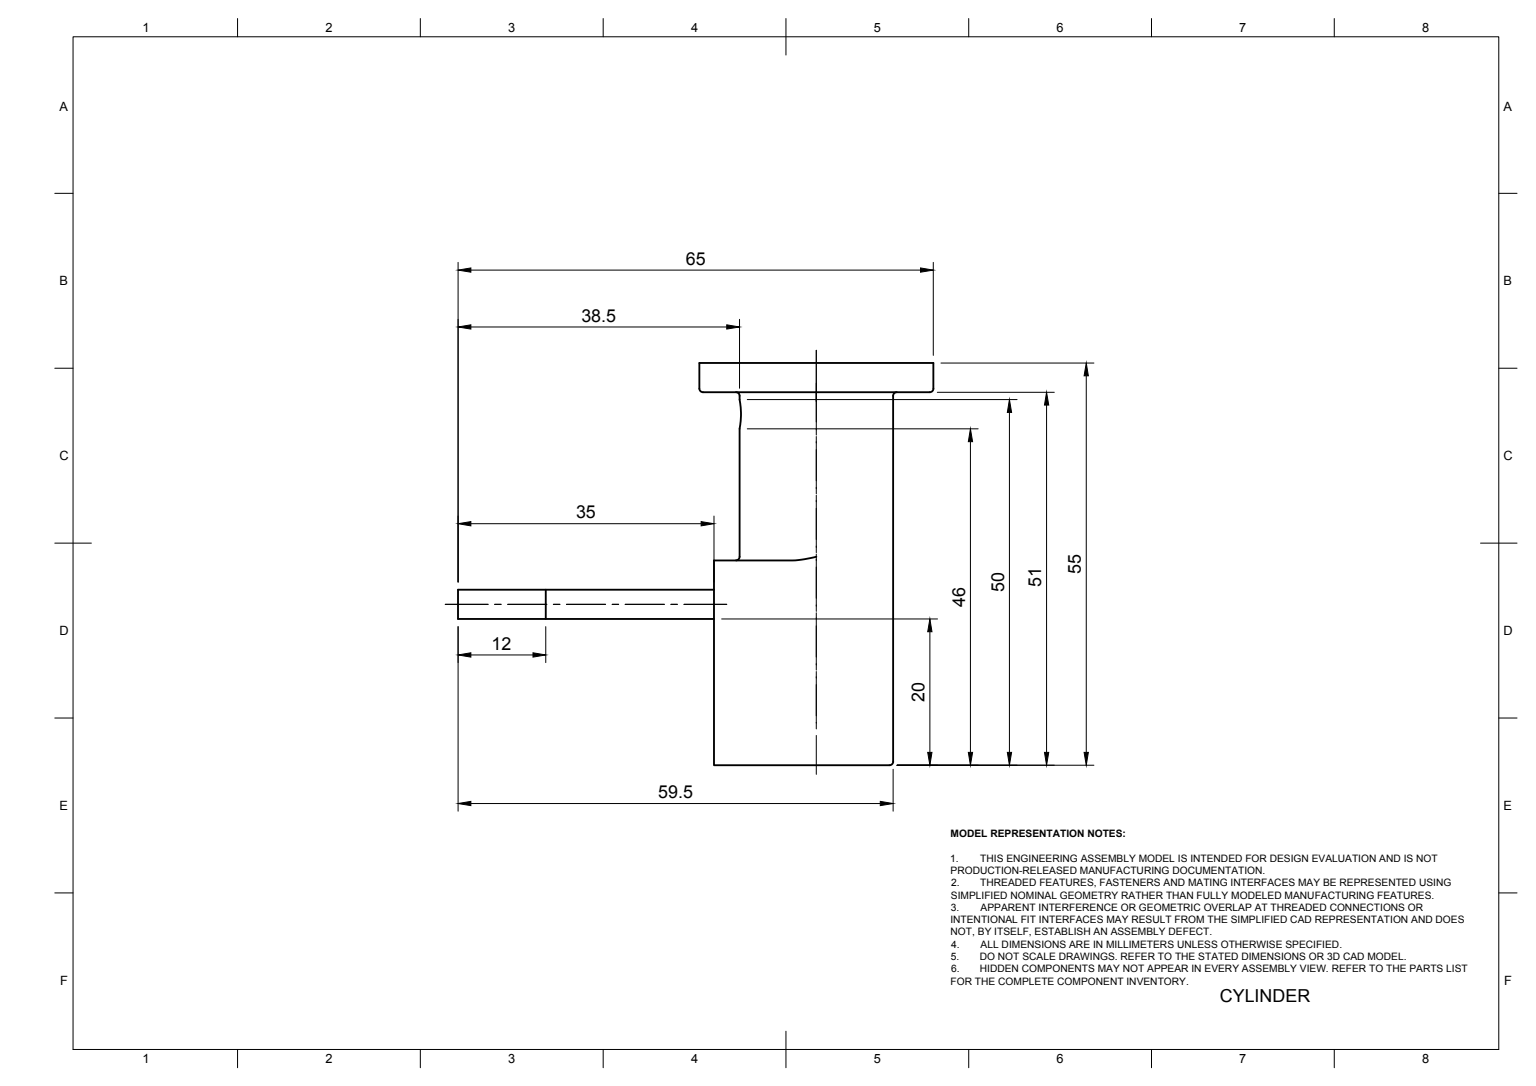
ISO-10303-21;
HEADER;
/* Generated by software containing ST-Developer
 * from STEP Tools, Inc. (www.steptools.com) 
 */

FILE_DESCRIPTION(
/* description */ (''),
/* implementation_level */ '2;1');

FILE_NAME(
/* name */ 'CYLINDER.step',
/* time_stamp */ '2026-10-06T01:16:10-07:00',
/* author */ (''),
/* organization */ (''),
/* preprocessor_version */ 'ST-DEVELOPER v20.2',
/* originating_system */ 'Autodesk Translation Framework v15.15.0.0',
/* authorisation */ '');

FILE_SCHEMA (('AUTOMOTIVE_DESIGN { 1 0 10303 214 3 1 1 }'));
ENDSEC;

DATA;
#10=MECHANICAL_DESIGN_GEOMETRIC_PRESENTATION_REPRESENTATION('',(#312,#313,#314,#315,#316,#317),#17113);
#138=TOROIDAL_SURFACE('',#6725,15.5,0.5);
#139=TOROIDAL_SURFACE('',#6736,11.,0.5);
#140=TOROIDAL_SURFACE('',#6744,10.9999999985,0.5);
#141=TOROIDAL_SURFACE('',#6748,10.,0.5);
#196=B_SPLINE_CURVE_WITH_KNOTS('',3,(#11224,#11225,#11226,#11227,#11228,
#11229,#11230,#11231,#11232,#11233,#11234,#11235,#11236,#11237,#11238,#11239,
#11240,#11241),.UNSPECIFIED.,.F.,.F.,(4,2,2,2,2,2,2,2,4),(-1.05841496918539,
-0.992261360989225,-0.926107752793056,-0.859959489841051,-0.793811226889045,
-0.72766296393704,-0.661514700985034,-0.595361092788865,-0.529207484592697),
 .UNSPECIFIED.);
#197=B_SPLINE_CURVE_WITH_KNOTS('',3,(#11242,#11243,#11244,#11245,#11246,
#11247,#11248,#11249,#11250,#11251,#11252,#11253,#11254,#11255,#11256,#11257,
#11258,#11259),.UNSPECIFIED.,.F.,.F.,(4,2,2,2,2,2,2,2,4),(-0.529207484592697,
-0.463053876396528,-0.39690026820036,-0.330752005248354,-0.264603742296348,
-0.198455479344343,-0.132307216392337,-0.0661536081961685,0.),
 .UNSPECIFIED.);
#198=B_SPLINE_CURVE_WITH_KNOTS('',3,(#11269,#11270,#11271,#11272,#11273,
#11274,#11275,#11276,#11277,#11278,#11279,#11280,#11281,#11282,#11283,#11284,
#11285,#11286),.UNSPECIFIED.,.F.,.F.,(4,2,2,2,2,2,2,2,4),(0.,0.0756896464070345,
0.151379292814069,0.227058356460011,0.302737420105953,0.378416483751896,
0.454095547397838,0.529785193804872,0.605474840211907),.UNSPECIFIED.);
#199=B_SPLINE_CURVE_WITH_KNOTS('',3,(#11287,#11288,#11289,#11290,#11291,
#11292,#11293,#11294,#11295,#11296,#11297,#11298,#11299,#11300,#11301,#11302,
#11303,#11304),.UNSPECIFIED.,.F.,.F.,(4,2,2,2,2,2,2,2,4),(0.605474840211907,
0.681164486618941,0.756854133025976,0.832533196671918,0.90821226031786,
0.983891323963802,1.05957038760974,1.13526003401678,1.21094968042381),
 .UNSPECIFIED.);
#200=B_SPLINE_CURVE_WITH_KNOTS('',3,(#11355,#11356,#11357,#11358,#11359,
#11360,#11361,#11362,#11363,#11364,#11365,#11366,#11367,#11368,#11369,#11370,
#11371,#11372,#11373,#11374,#11375,#11376,#11377,#11378,#11379,#11380,#11381,
#11382,#11383,#11384,#11385,#11386,#11387,#11388),.UNSPECIFIED.,.T.,.F.,
(4,2,2,2,2,2,2,2,2,2,2,2,2,2,2,2,4),(-1.20857841771805,-1.13304053166828,
-1.05750264561851,-0.981968229453524,-0.906433813288534,-0.830899397123545,
-0.755364980958556,-0.679827094908789,-0.604289208859023,-0.528751322809257,
-0.45321343675949,-0.377679020594501,-0.302144604429511,-0.226610188264522,
-0.151075772099533,-0.0755378860497663,0.),.UNSPECIFIED.);
#201=B_SPLINE_CURVE_WITH_KNOTS('',3,(#11395,#11396,#11397,#11398),
 .UNSPECIFIED.,.F.,.F.,(4,4),(2.52799303913365E-15,0.312557295914921),
 .UNSPECIFIED.);
#202=B_SPLINE_CURVE_WITH_KNOTS('',3,(#11399,#11400,#11401,#11402),
 .UNSPECIFIED.,.F.,.F.,(4,4),(0.616643793973297,0.929201089887433),
 .UNSPECIFIED.);
#229=OPEN_SHELL('',(#5914,#5915));
#230=OPEN_SHELL('',(#5916,#5917));
#231=OPEN_SHELL('',(#5918,#5919));
#232=OPEN_SHELL('',(#5920,#5921));
#233=OPEN_SHELL('',(#5922,#5923));
#247=SHELL_BASED_SURFACE_MODEL('Body2',(#229));
#248=SHELL_BASED_SURFACE_MODEL('Body3',(#230));
#249=SHELL_BASED_SURFACE_MODEL('Body4',(#231));
#250=SHELL_BASED_SURFACE_MODEL('Body5',(#232));
#251=SHELL_BASED_SURFACE_MODEL('Body6',(#233));
#272=SHAPE_REPRESENTATION_RELATIONSHIP('SRR','None',#17197,#288);
#288=ADVANCED_BREP_SHAPE_REPRESENTATION('',(#338),#17104);
#312=STYLED_ITEM('',(#17298),#338);
#313=STYLED_ITEM('',(#17298),#247);
#314=STYLED_ITEM('',(#17298),#248);
#315=STYLED_ITEM('',(#17298),#249);
#316=STYLED_ITEM('',(#17298),#250);
#317=STYLED_ITEM('',(#17298),#251);
#338=MANIFOLD_SOLID_BREP('Body1',#6024);
#450=CYLINDRICAL_SURFACE('',#6706,0.5);
#451=CYLINDRICAL_SURFACE('',#6713,1.75);
#452=CYLINDRICAL_SURFACE('',#6714,8.);
#453=CYLINDRICAL_SURFACE('',#6722,16.);
#454=CYLINDRICAL_SURFACE('',#6733,1.25);
#455=CYLINDRICAL_SURFACE('',#6734,1.25);
#456=CYLINDRICAL_SURFACE('',#6735,1.25);
#457=CYLINDRICAL_SURFACE('',#6740,10.5);
#458=CYLINDRICAL_SURFACE('',#6743,2.);
#459=CYLINDRICAL_SURFACE('',#6750,0.5);
#460=CYLINDRICAL_SURFACE('',#6753,2.);
#461=CYLINDRICAL_SURFACE('',#6756,1.5);
#462=CYLINDRICAL_SURFACE('',#6761,1.5);
#463=CYLINDRICAL_SURFACE('',#6766,1.5);
#464=CYLINDRICAL_SURFACE('',#6771,1.5);
#465=CYLINDRICAL_SURFACE('',#6776,1.75);
#588=FACE_BOUND('',#1689,.T.);
#589=FACE_BOUND('',#1690,.T.);
#590=FACE_BOUND('',#1693,.T.);
#591=FACE_BOUND('',#1694,.T.);
#592=FACE_BOUND('',#1696,.T.);
#593=FACE_BOUND('',#1697,.T.);
#594=FACE_BOUND('',#1698,.T.);
#595=FACE_BOUND('',#1699,.T.);
#596=FACE_BOUND('',#1703,.T.);
#597=FACE_BOUND('',#1704,.T.);
#598=FACE_BOUND('',#1705,.T.);
#599=FACE_BOUND('',#1706,.T.);
#600=FACE_BOUND('',#1712,.T.);
#601=FACE_BOUND('',#1725,.T.);
#602=FACE_BOUND('',#1728,.T.);
#603=FACE_BOUND('',#1731,.T.);
#604=FACE_BOUND('',#1734,.T.);
#605=FACE_BOUND('',#1737,.T.);
#875=CIRCLE('',#6705,10.);
#876=CIRCLE('',#6707,0.5);
#877=CIRCLE('',#6708,0.5);
#878=CIRCLE('',#6710,0.5);
#879=CIRCLE('',#6711,2.);
#880=CIRCLE('',#6712,1.75);
#881=CIRCLE('',#6715,8.);
#882=CIRCLE('',#6716,8.);
#883=CIRCLE('',#6718,16.);
#884=CIRCLE('',#6719,1.25);
#885=CIRCLE('',#6720,1.25);
#886=CIRCLE('',#6721,1.25);
#887=CIRCLE('',#6723,16.);
#888=CIRCLE('',#6724,16.);
#889=CIRCLE('',#6726,0.5);
#890=CIRCLE('',#6727,15.5);
#891=CIRCLE('',#6729,1.25);
#892=CIRCLE('',#6730,1.25);
#893=CIRCLE('',#6731,11.);
#894=CIRCLE('',#6732,1.25);
#895=CIRCLE('',#6737,0.5);
#896=CIRCLE('',#6738,10.5);
#897=CIRCLE('',#6739,10.5);
#898=CIRCLE('',#6741,10.4999999985);
#899=CIRCLE('',#6742,10.5);
#900=CIRCLE('',#6745,10.9999999985);
#901=CIRCLE('',#6749,0.5);
#902=CIRCLE('',#6754,2.);
#903=CIRCLE('',#6757,1.5);
#904=CIRCLE('',#6758,1.5);
#905=CIRCLE('',#6760,1.25);
#906=CIRCLE('',#6762,1.5);
#907=CIRCLE('',#6763,1.5);
#908=CIRCLE('',#6765,1.25);
#909=CIRCLE('',#6767,1.5);
#910=CIRCLE('',#6768,1.5);
#911=CIRCLE('',#6770,1.25);
#912=CIRCLE('',#6772,1.5);
#913=CIRCLE('',#6773,1.5);
#914=CIRCLE('',#6775,1.25);
#915=CIRCLE('',#6777,1.75);
#916=CIRCLE('',#6778,1.75);
#917=CIRCLE('',#6780,2.);
#1242=FACE_OUTER_BOUND('',#1686,.T.);
#1243=FACE_OUTER_BOUND('',#1687,.T.);
#1244=FACE_OUTER_BOUND('',#1688,.T.);
#1245=FACE_OUTER_BOUND('',#1691,.T.);
#1246=FACE_OUTER_BOUND('',#1692,.T.);
#1247=FACE_OUTER_BOUND('',#1695,.T.);
#1248=FACE_OUTER_BOUND('',#1700,.T.);
#1249=FACE_OUTER_BOUND('',#1701,.T.);
#1250=FACE_OUTER_BOUND('',#1702,.T.);
#1251=FACE_OUTER_BOUND('',#1707,.T.);
#1252=FACE_OUTER_BOUND('',#1708,.T.);
#1253=FACE_OUTER_BOUND('',#1709,.T.);
#1254=FACE_OUTER_BOUND('',#1710,.T.);
#1255=FACE_OUTER_BOUND('',#1711,.T.);
#1256=FACE_OUTER_BOUND('',#1713,.T.);
#1257=FACE_OUTER_BOUND('',#1714,.T.);
#1258=FACE_OUTER_BOUND('',#1715,.T.);
#1259=FACE_OUTER_BOUND('',#1716,.T.);
#1260=FACE_OUTER_BOUND('',#1717,.T.);
#1261=FACE_OUTER_BOUND('',#1718,.T.);
#1262=FACE_OUTER_BOUND('',#1719,.T.);
#1263=FACE_OUTER_BOUND('',#1720,.T.);
#1264=FACE_OUTER_BOUND('',#1721,.T.);
#1265=FACE_OUTER_BOUND('',#1722,.T.);
#1266=FACE_OUTER_BOUND('',#1723,.T.);
#1267=FACE_OUTER_BOUND('',#1724,.T.);
#1268=FACE_OUTER_BOUND('',#1726,.T.);
#1269=FACE_OUTER_BOUND('',#1727,.T.);
#1270=FACE_OUTER_BOUND('',#1729,.T.);
#1271=FACE_OUTER_BOUND('',#1730,.T.);
#1272=FACE_OUTER_BOUND('',#1732,.T.);
#1273=FACE_OUTER_BOUND('',#1733,.T.);
#1274=FACE_OUTER_BOUND('',#1735,.T.);
#1275=FACE_OUTER_BOUND('',#1736,.T.);
#1686=EDGE_LOOP('',(#4980,#4981,#4982,#4983));
#1687=EDGE_LOOP('',(#4984,#4985,#4986,#4987));
#1688=EDGE_LOOP('',(#4988,#4989,#4990,#4991,#4992,#4993));
#1689=EDGE_LOOP('',(#4994));
#1690=EDGE_LOOP('',(#4995));
#1691=EDGE_LOOP('',(#4996,#4997,#4998,#4999,#5000));
#1692=EDGE_LOOP('',(#5001,#5002,#5003,#5004));
#1693=EDGE_LOOP('',(#5005,#5006));
#1694=EDGE_LOOP('',(#5007,#5008));
#1695=EDGE_LOOP('',(#5009));
#1696=EDGE_LOOP('',(#5010));
#1697=EDGE_LOOP('',(#5011));
#1698=EDGE_LOOP('',(#5012));
#1699=EDGE_LOOP('',(#5013));
#1700=EDGE_LOOP('',(#5014,#5015,#5016,#5017,#5018));
#1701=EDGE_LOOP('',(#5019,#5020,#5021,#5022,#5023));
#1702=EDGE_LOOP('',(#5024));
#1703=EDGE_LOOP('',(#5025));
#1704=EDGE_LOOP('',(#5026));
#1705=EDGE_LOOP('',(#5027));
#1706=EDGE_LOOP('',(#5028));
#1707=EDGE_LOOP('',(#5029,#5030,#5031,#5032));
#1708=EDGE_LOOP('',(#5033,#5034,#5035,#5036));
#1709=EDGE_LOOP('',(#5037,#5038,#5039,#5040));
#1710=EDGE_LOOP('',(#5041,#5042,#5043,#5044,#5045));
#1711=EDGE_LOOP('',(#5046,#5047,#5048,#5049,#5050,#5051,#5052,#5053));
#1712=EDGE_LOOP('',(#5054));
#1713=EDGE_LOOP('',(#5055,#5056,#5057,#5058,#5059));
#1714=EDGE_LOOP('',(#5060,#5061,#5062,#5063));
#1715=EDGE_LOOP('',(#5064,#5065,#5066,#5067));
#1716=EDGE_LOOP('',(#5068,#5069,#5070,#5071,#5072));
#1717=EDGE_LOOP('',(#5073,#5074,#5075,#5076));
#1718=EDGE_LOOP('',(#5077,#5078,#5079,#5080));
#1719=EDGE_LOOP('',(#5081,#5082,#5083,#5084,#5085));
#1720=EDGE_LOOP('',(#5086));
#1721=EDGE_LOOP('',(#5087,#5088,#5089,#5090));
#1722=EDGE_LOOP('',(#5091));
#1723=EDGE_LOOP('',(#5092,#5093,#5094,#5095));
#1724=EDGE_LOOP('',(#5096));
#1725=EDGE_LOOP('',(#5097));
#1726=EDGE_LOOP('',(#5098,#5099,#5100,#5101));
#1727=EDGE_LOOP('',(#5102));
#1728=EDGE_LOOP('',(#5103));
#1729=EDGE_LOOP('',(#5104,#5105,#5106,#5107));
#1730=EDGE_LOOP('',(#5108));
#1731=EDGE_LOOP('',(#5109));
#1732=EDGE_LOOP('',(#5110,#5111,#5112,#5113));
#1733=EDGE_LOOP('',(#5114));
#1734=EDGE_LOOP('',(#5115));
#1735=EDGE_LOOP('',(#5116,#5117,#5118,#5119));
#1736=EDGE_LOOP('',(#5120));
#1737=EDGE_LOOP('',(#5121));
#2107=LINE('',#11197,#2468);
#2108=LINE('',#11199,#2469);
#2109=LINE('',#11201,#2470);
#2110=LINE('',#11208,#2471);
#2111=LINE('',#11211,#2472);
#2112=LINE('',#11213,#2473);
#2113=LINE('',#11215,#2474);
#2114=LINE('',#11260,#2475);
#2115=LINE('',#11265,#2476);
#2116=LINE('',#11316,#2477);
#2117=LINE('',#11334,#2478);
#2118=LINE('',#11336,#2479);
#2119=LINE('',#11338,#2480);
#2120=LINE('',#11347,#2481);
#2121=LINE('',#11350,#2482);
#2122=LINE('',#11353,#2483);
#2123=LINE('',#11390,#2484);
#2124=LINE('',#11404,#2485);
#2125=LINE('',#11405,#2486);
#2126=LINE('',#11410,#2487);
#2127=LINE('',#11416,#2488);
#2128=LINE('',#11422,#2489);
#2129=LINE('',#11431,#2490);
#2130=LINE('',#11440,#2491);
#2131=LINE('',#11449,#2492);
#2132=LINE('',#11458,#2493);
#2468=VECTOR('',#8217,14.);
#2469=VECTOR('',#8218,20.);
#2470=VECTOR('',#8219,14.);
#2471=VECTOR('',#8228,13.99999999978);
#2472=VECTOR('',#8231,27.5);
#2473=VECTOR('',#8232,21.);
#2474=VECTOR('',#8233,27.5);
#2475=VECTOR('',#8242,1.75);
#2476=VECTOR('',#8247,8.);
#2477=VECTOR('',#8262,16.);
#2478=VECTOR('',#8285,1.25);
#2479=VECTOR('',#8288,1.25);
#2480=VECTOR('',#8291,1.25);
#2481=VECTOR('',#8302,10.5);
#2482=VECTOR('',#8305,28.);
#2483=VECTOR('',#8308,28.);
#2484=VECTOR('',#8311,2.);
#2485=VECTOR('',#8318,10.72128073786);
#2486=VECTOR('',#8319,10.72128073785);
#2487=VECTOR('',#8328,13.9999999992);
#2488=VECTOR('',#8337,2.);
#2489=VECTOR('',#8344,1.5);
#2490=VECTOR('',#8355,1.5);
#2491=VECTOR('',#8366,1.5);
#2492=VECTOR('',#8377,1.5);
#2493=VECTOR('',#8388,1.75);
#2922=VERTEX_POINT('',#11195);
#2923=VERTEX_POINT('',#11196);
#2924=VERTEX_POINT('',#11198);
#2925=VERTEX_POINT('',#11200);
#2926=VERTEX_POINT('',#11204);
#2927=VERTEX_POINT('',#11206);
#2928=VERTEX_POINT('',#11210);
#2929=VERTEX_POINT('',#11212);
#2930=VERTEX_POINT('',#11214);
#2931=VERTEX_POINT('',#11217);
#2932=VERTEX_POINT('',#11219);
#2933=VERTEX_POINT('',#11222);
#2934=VERTEX_POINT('',#11223);
#2935=VERTEX_POINT('',#11262);
#2936=VERTEX_POINT('',#11264);
#2937=VERTEX_POINT('',#11267);
#2938=VERTEX_POINT('',#11268);
#2939=VERTEX_POINT('',#11306);
#2940=VERTEX_POINT('',#11308);
#2941=VERTEX_POINT('',#11310);
#2942=VERTEX_POINT('',#11312);
#2943=VERTEX_POINT('',#11315);
#2944=VERTEX_POINT('',#11317);
#2945=VERTEX_POINT('',#11321);
#2946=VERTEX_POINT('',#11325);
#2947=VERTEX_POINT('',#11327);
#2948=VERTEX_POINT('',#11329);
#2949=VERTEX_POINT('',#11331);
#2950=VERTEX_POINT('',#11340);
#2951=VERTEX_POINT('',#11342);
#2952=VERTEX_POINT('',#11346);
#2953=VERTEX_POINT('',#11348);
#2954=VERTEX_POINT('',#11351);
#2955=VERTEX_POINT('',#11354);
#2956=VERTEX_POINT('',#11392);
#2957=VERTEX_POINT('',#11393);
#2958=VERTEX_POINT('',#11414);
#2959=VERTEX_POINT('',#11419);
#2960=VERTEX_POINT('',#11421);
#2961=VERTEX_POINT('',#11425);
#2962=VERTEX_POINT('',#11428);
#2963=VERTEX_POINT('',#11430);
#2964=VERTEX_POINT('',#11434);
#2965=VERTEX_POINT('',#11437);
#2966=VERTEX_POINT('',#11439);
#2967=VERTEX_POINT('',#11443);
#2968=VERTEX_POINT('',#11446);
#2969=VERTEX_POINT('',#11448);
#2970=VERTEX_POINT('',#11452);
#2971=VERTEX_POINT('',#11455);
#2972=VERTEX_POINT('',#11457);
#2973=VERTEX_POINT('',#11461);
#3644=EDGE_CURVE('',#2922,#2923,#2107,.T.);
#3645=EDGE_CURVE('',#2924,#2923,#2108,.T.);
#3646=EDGE_CURVE('',#2924,#2925,#2109,.T.);
#3647=EDGE_CURVE('',#2925,#2922,#875,.T.);
#3648=EDGE_CURVE('',#2923,#2926,#876,.T.);
#3649=EDGE_CURVE('',#2922,#2927,#877,.T.);
#3650=EDGE_CURVE('',#2927,#2926,#2110,.T.);
#3651=EDGE_CURVE('',#2926,#2928,#2111,.T.);
#3652=EDGE_CURVE('',#2928,#2929,#2112,.T.);
#3653=EDGE_CURVE('',#2929,#2930,#2113,.T.);
#3654=EDGE_CURVE('',#2930,#2924,#878,.T.);
#3655=EDGE_CURVE('',#2931,#2931,#879,.T.);
#3656=EDGE_CURVE('',#2932,#2932,#880,.T.);
#3657=EDGE_CURVE('',#2933,#2934,#196,.T.);
#3658=EDGE_CURVE('',#2934,#2933,#197,.T.);
#3659=EDGE_CURVE('',#2934,#2932,#2114,.T.);
#3660=EDGE_CURVE('',#2935,#2935,#881,.T.);
#3661=EDGE_CURVE('',#2935,#2936,#2115,.T.);
#3662=EDGE_CURVE('',#2936,#2936,#882,.T.);
#3663=EDGE_CURVE('',#2937,#2938,#198,.T.);
#3664=EDGE_CURVE('',#2938,#2937,#199,.T.);
#3665=EDGE_CURVE('',#2939,#2939,#883,.T.);
#3666=EDGE_CURVE('',#2940,#2940,#884,.T.);
#3667=EDGE_CURVE('',#2941,#2941,#885,.T.);
#3668=EDGE_CURVE('',#2942,#2942,#886,.T.);
#3669=EDGE_CURVE('',#2939,#2943,#2116,.T.);
#3670=EDGE_CURVE('',#2943,#2944,#887,.T.);
#3671=EDGE_CURVE('',#2944,#2943,#888,.T.);
#3672=EDGE_CURVE('',#2944,#2945,#889,.T.);
#3673=EDGE_CURVE('',#2945,#2945,#890,.T.);
#3674=EDGE_CURVE('',#2946,#2946,#891,.T.);
#3675=EDGE_CURVE('',#2947,#2947,#892,.T.);
#3676=EDGE_CURVE('',#2948,#2948,#893,.T.);
#3677=EDGE_CURVE('',#2949,#2949,#894,.T.);
#3678=EDGE_CURVE('',#2949,#2940,#2117,.T.);
#3679=EDGE_CURVE('',#2946,#2941,#2118,.T.);
#3680=EDGE_CURVE('',#2947,#2942,#2119,.T.);
#3681=EDGE_CURVE('',#2948,#2950,#895,.T.);
#3682=EDGE_CURVE('',#2951,#2950,#896,.T.);
#3683=EDGE_CURVE('',#2950,#2951,#897,.T.);
#3684=EDGE_CURVE('',#2951,#2952,#2120,.T.);
#3685=EDGE_CURVE('',#2952,#2953,#898,.T.);
#3686=EDGE_CURVE('',#2953,#2927,#2121,.T.);
#3687=EDGE_CURVE('',#2954,#2927,#899,.T.);
#3688=EDGE_CURVE('',#2954,#2952,#2122,.T.);
#3689=EDGE_CURVE('',#2955,#2955,#200,.T.);
#3690=EDGE_CURVE('',#2938,#2955,#2123,.T.);
#3691=EDGE_CURVE('',#2956,#2957,#900,.T.);
#3692=EDGE_CURVE('',#2953,#2956,#201,.T.);
#3693=EDGE_CURVE('',#2957,#2952,#202,.T.);
#3694=EDGE_CURVE('',#2929,#2957,#2124,.T.);
#3695=EDGE_CURVE('',#2928,#2956,#2125,.T.);
#3696=EDGE_CURVE('',#2925,#2954,#901,.T.);
#3697=EDGE_CURVE('',#2930,#2954,#2126,.T.);
#3698=EDGE_CURVE('',#2958,#2958,#902,.T.);
#3699=EDGE_CURVE('',#2958,#2931,#2127,.T.);
#3700=EDGE_CURVE('',#2959,#2959,#903,.T.);
#3701=EDGE_CURVE('',#2959,#2960,#2128,.T.);
#3702=EDGE_CURVE('',#2960,#2960,#904,.T.);
#3703=EDGE_CURVE('',#2961,#2961,#905,.T.);
#3704=EDGE_CURVE('',#2962,#2962,#906,.T.);
#3705=EDGE_CURVE('',#2962,#2963,#2129,.T.);
#3706=EDGE_CURVE('',#2963,#2963,#907,.T.);
#3707=EDGE_CURVE('',#2964,#2964,#908,.T.);
#3708=EDGE_CURVE('',#2965,#2965,#909,.T.);
#3709=EDGE_CURVE('',#2965,#2966,#2130,.T.);
#3710=EDGE_CURVE('',#2966,#2966,#910,.T.);
#3711=EDGE_CURVE('',#2967,#2967,#911,.T.);
#3712=EDGE_CURVE('',#2968,#2968,#912,.T.);
#3713=EDGE_CURVE('',#2968,#2969,#2131,.T.);
#3714=EDGE_CURVE('',#2969,#2969,#913,.T.);
#3715=EDGE_CURVE('',#2970,#2970,#914,.T.);
#3716=EDGE_CURVE('',#2971,#2971,#915,.T.);
#3717=EDGE_CURVE('',#2971,#2972,#2132,.T.);
#3718=EDGE_CURVE('',#2972,#2972,#916,.T.);
#3719=EDGE_CURVE('',#2973,#2973,#917,.T.);
#4980=ORIENTED_EDGE('',*,*,#3644,.T.);
#4981=ORIENTED_EDGE('',*,*,#3645,.F.);
#4982=ORIENTED_EDGE('',*,*,#3646,.T.);
#4983=ORIENTED_EDGE('',*,*,#3647,.T.);
#4984=ORIENTED_EDGE('',*,*,#3648,.F.);
#4985=ORIENTED_EDGE('',*,*,#3644,.F.);
#4986=ORIENTED_EDGE('',*,*,#3649,.T.);
#4987=ORIENTED_EDGE('',*,*,#3650,.T.);
#4988=ORIENTED_EDGE('',*,*,#3648,.T.);
#4989=ORIENTED_EDGE('',*,*,#3651,.T.);
#4990=ORIENTED_EDGE('',*,*,#3652,.T.);
#4991=ORIENTED_EDGE('',*,*,#3653,.T.);
#4992=ORIENTED_EDGE('',*,*,#3654,.T.);
#4993=ORIENTED_EDGE('',*,*,#3645,.T.);
#4994=ORIENTED_EDGE('',*,*,#3655,.F.);
#4995=ORIENTED_EDGE('',*,*,#3656,.F.);
#4996=ORIENTED_EDGE('',*,*,#3657,.F.);
#4997=ORIENTED_EDGE('',*,*,#3658,.F.);
#4998=ORIENTED_EDGE('',*,*,#3659,.T.);
#4999=ORIENTED_EDGE('',*,*,#3656,.T.);
#5000=ORIENTED_EDGE('',*,*,#3659,.F.);
#5001=ORIENTED_EDGE('',*,*,#3660,.F.);
#5002=ORIENTED_EDGE('',*,*,#3661,.T.);
#5003=ORIENTED_EDGE('',*,*,#3662,.T.);
#5004=ORIENTED_EDGE('',*,*,#3661,.F.);
#5005=ORIENTED_EDGE('',*,*,#3657,.T.);
#5006=ORIENTED_EDGE('',*,*,#3658,.T.);
#5007=ORIENTED_EDGE('',*,*,#3663,.T.);
#5008=ORIENTED_EDGE('',*,*,#3664,.T.);
#5009=ORIENTED_EDGE('',*,*,#3665,.F.);
#5010=ORIENTED_EDGE('',*,*,#3662,.F.);
#5011=ORIENTED_EDGE('',*,*,#3666,.F.);
#5012=ORIENTED_EDGE('',*,*,#3667,.F.);
#5013=ORIENTED_EDGE('',*,*,#3668,.F.);
#5014=ORIENTED_EDGE('',*,*,#3665,.T.);
#5015=ORIENTED_EDGE('',*,*,#3669,.T.);
#5016=ORIENTED_EDGE('',*,*,#3670,.T.);
#5017=ORIENTED_EDGE('',*,*,#3671,.T.);
#5018=ORIENTED_EDGE('',*,*,#3669,.F.);
#5019=ORIENTED_EDGE('',*,*,#3670,.F.);
#5020=ORIENTED_EDGE('',*,*,#3671,.F.);
#5021=ORIENTED_EDGE('',*,*,#3672,.T.);
#5022=ORIENTED_EDGE('',*,*,#3673,.T.);
#5023=ORIENTED_EDGE('',*,*,#3672,.F.);
#5024=ORIENTED_EDGE('',*,*,#3673,.F.);
#5025=ORIENTED_EDGE('',*,*,#3674,.T.);
#5026=ORIENTED_EDGE('',*,*,#3675,.T.);
#5027=ORIENTED_EDGE('',*,*,#3676,.F.);
#5028=ORIENTED_EDGE('',*,*,#3677,.T.);
#5029=ORIENTED_EDGE('',*,*,#3677,.F.);
#5030=ORIENTED_EDGE('',*,*,#3678,.T.);
#5031=ORIENTED_EDGE('',*,*,#3666,.T.);
#5032=ORIENTED_EDGE('',*,*,#3678,.F.);
#5033=ORIENTED_EDGE('',*,*,#3674,.F.);
#5034=ORIENTED_EDGE('',*,*,#3679,.T.);
#5035=ORIENTED_EDGE('',*,*,#3667,.T.);
#5036=ORIENTED_EDGE('',*,*,#3679,.F.);
#5037=ORIENTED_EDGE('',*,*,#3675,.F.);
#5038=ORIENTED_EDGE('',*,*,#3680,.T.);
#5039=ORIENTED_EDGE('',*,*,#3668,.T.);
#5040=ORIENTED_EDGE('',*,*,#3680,.F.);
#5041=ORIENTED_EDGE('',*,*,#3676,.T.);
#5042=ORIENTED_EDGE('',*,*,#3681,.T.);
#5043=ORIENTED_EDGE('',*,*,#3682,.F.);
#5044=ORIENTED_EDGE('',*,*,#3683,.F.);
#5045=ORIENTED_EDGE('',*,*,#3681,.F.);
#5046=ORIENTED_EDGE('',*,*,#3682,.T.);
#5047=ORIENTED_EDGE('',*,*,#3683,.T.);
#5048=ORIENTED_EDGE('',*,*,#3684,.T.);
#5049=ORIENTED_EDGE('',*,*,#3685,.T.);
#5050=ORIENTED_EDGE('',*,*,#3686,.T.);
#5051=ORIENTED_EDGE('',*,*,#3687,.F.);
#5052=ORIENTED_EDGE('',*,*,#3688,.T.);
#5053=ORIENTED_EDGE('',*,*,#3684,.F.);
#5054=ORIENTED_EDGE('',*,*,#3689,.T.);
#5055=ORIENTED_EDGE('',*,*,#3663,.F.);
#5056=ORIENTED_EDGE('',*,*,#3664,.F.);
#5057=ORIENTED_EDGE('',*,*,#3690,.T.);
#5058=ORIENTED_EDGE('',*,*,#3689,.F.);
#5059=ORIENTED_EDGE('',*,*,#3690,.F.);
#5060=ORIENTED_EDGE('',*,*,#3691,.F.);
#5061=ORIENTED_EDGE('',*,*,#3692,.F.);
#5062=ORIENTED_EDGE('',*,*,#3685,.F.);
#5063=ORIENTED_EDGE('',*,*,#3693,.F.);
#5064=ORIENTED_EDGE('',*,*,#3691,.T.);
#5065=ORIENTED_EDGE('',*,*,#3694,.F.);
#5066=ORIENTED_EDGE('',*,*,#3652,.F.);
#5067=ORIENTED_EDGE('',*,*,#3695,.T.);
#5068=ORIENTED_EDGE('',*,*,#3650,.F.);
#5069=ORIENTED_EDGE('',*,*,#3686,.F.);
#5070=ORIENTED_EDGE('',*,*,#3692,.T.);
#5071=ORIENTED_EDGE('',*,*,#3695,.F.);
#5072=ORIENTED_EDGE('',*,*,#3651,.F.);
#5073=ORIENTED_EDGE('',*,*,#3647,.F.);
#5074=ORIENTED_EDGE('',*,*,#3696,.T.);
#5075=ORIENTED_EDGE('',*,*,#3687,.T.);
#5076=ORIENTED_EDGE('',*,*,#3649,.F.);
#5077=ORIENTED_EDGE('',*,*,#3654,.F.);
#5078=ORIENTED_EDGE('',*,*,#3697,.T.);
#5079=ORIENTED_EDGE('',*,*,#3696,.F.);
#5080=ORIENTED_EDGE('',*,*,#3646,.F.);
#5081=ORIENTED_EDGE('',*,*,#3697,.F.);
#5082=ORIENTED_EDGE('',*,*,#3653,.F.);
#5083=ORIENTED_EDGE('',*,*,#3694,.T.);
#5084=ORIENTED_EDGE('',*,*,#3693,.T.);
#5085=ORIENTED_EDGE('',*,*,#3688,.F.);
#5086=ORIENTED_EDGE('',*,*,#3660,.T.);
#5087=ORIENTED_EDGE('',*,*,#3698,.F.);
#5088=ORIENTED_EDGE('',*,*,#3699,.T.);
#5089=ORIENTED_EDGE('',*,*,#3655,.T.);
#5090=ORIENTED_EDGE('',*,*,#3699,.F.);
#5091=ORIENTED_EDGE('',*,*,#3698,.T.);
#5092=ORIENTED_EDGE('',*,*,#3700,.F.);
#5093=ORIENTED_EDGE('',*,*,#3701,.T.);
#5094=ORIENTED_EDGE('',*,*,#3702,.T.);
#5095=ORIENTED_EDGE('',*,*,#3701,.F.);
#5096=ORIENTED_EDGE('',*,*,#3702,.F.);
#5097=ORIENTED_EDGE('',*,*,#3703,.F.);
#5098=ORIENTED_EDGE('',*,*,#3704,.F.);
#5099=ORIENTED_EDGE('',*,*,#3705,.T.);
#5100=ORIENTED_EDGE('',*,*,#3706,.T.);
#5101=ORIENTED_EDGE('',*,*,#3705,.F.);
#5102=ORIENTED_EDGE('',*,*,#3706,.F.);
#5103=ORIENTED_EDGE('',*,*,#3707,.F.);
#5104=ORIENTED_EDGE('',*,*,#3708,.F.);
#5105=ORIENTED_EDGE('',*,*,#3709,.T.);
#5106=ORIENTED_EDGE('',*,*,#3710,.T.);
#5107=ORIENTED_EDGE('',*,*,#3709,.F.);
#5108=ORIENTED_EDGE('',*,*,#3710,.F.);
#5109=ORIENTED_EDGE('',*,*,#3711,.F.);
#5110=ORIENTED_EDGE('',*,*,#3712,.F.);
#5111=ORIENTED_EDGE('',*,*,#3713,.T.);
#5112=ORIENTED_EDGE('',*,*,#3714,.T.);
#5113=ORIENTED_EDGE('',*,*,#3713,.F.);
#5114=ORIENTED_EDGE('',*,*,#3714,.F.);
#5115=ORIENTED_EDGE('',*,*,#3715,.F.);
#5116=ORIENTED_EDGE('',*,*,#3716,.F.);
#5117=ORIENTED_EDGE('',*,*,#3717,.T.);
#5118=ORIENTED_EDGE('',*,*,#3718,.T.);
#5119=ORIENTED_EDGE('',*,*,#3717,.F.);
#5120=ORIENTED_EDGE('',*,*,#3719,.F.);
#5121=ORIENTED_EDGE('',*,*,#3718,.F.);
#5598=PLANE('',#6704);
#5599=PLANE('',#6709);
#5600=PLANE('',#6717);
#5601=PLANE('',#6728);
#5602=PLANE('',#6746);
#5603=PLANE('',#6747);
#5604=PLANE('',#6751);
#5605=PLANE('',#6752);
#5606=PLANE('',#6755);
#5607=PLANE('',#6759);
#5608=PLANE('',#6764);
#5609=PLANE('',#6769);
#5610=PLANE('',#6774);
#5611=PLANE('',#6779);
#5890=ADVANCED_FACE('',(#1242),#5598,.F.);
#5891=ADVANCED_FACE('',(#1243),#450,.T.);
#5892=ADVANCED_FACE('',(#1244,#588,#589),#5599,.T.);
#5893=ADVANCED_FACE('',(#1245),#451,.F.);
#5894=ADVANCED_FACE('',(#1246,#590,#591),#452,.F.);
#5895=ADVANCED_FACE('',(#1247,#592,#593,#594,#595),#5600,.T.);
#5896=ADVANCED_FACE('',(#1248),#453,.T.);
#5897=ADVANCED_FACE('',(#1249),#138,.T.);
#5898=ADVANCED_FACE('',(#1250,#596,#597,#598,#599),#5601,.F.);
#5899=ADVANCED_FACE('',(#1251),#454,.F.);
#5900=ADVANCED_FACE('',(#1252),#455,.F.);
#5901=ADVANCED_FACE('',(#1253),#456,.F.);
#5902=ADVANCED_FACE('',(#1254),#139,.F.);
#5903=ADVANCED_FACE('',(#1255,#600),#457,.T.);
#5904=ADVANCED_FACE('',(#1256),#458,.F.);
#5905=ADVANCED_FACE('',(#1257),#140,.F.);
#5906=ADVANCED_FACE('',(#1258),#5602,.T.);
#5907=ADVANCED_FACE('',(#1259),#5603,.T.);
#5908=ADVANCED_FACE('',(#1260),#141,.T.);
#5909=ADVANCED_FACE('',(#1261),#459,.T.);
#5910=ADVANCED_FACE('',(#1262),#5604,.T.);
#5911=ADVANCED_FACE('',(#1263),#5605,.T.);
#5912=ADVANCED_FACE('',(#1264),#460,.T.);
#5913=ADVANCED_FACE('',(#1265),#5606,.T.);
#5914=ADVANCED_FACE('',(#1266),#461,.T.);
#5915=ADVANCED_FACE('',(#1267,#601),#5607,.F.);
#5916=ADVANCED_FACE('',(#1268),#462,.T.);
#5917=ADVANCED_FACE('',(#1269,#602),#5608,.F.);
#5918=ADVANCED_FACE('',(#1270),#463,.T.);
#5919=ADVANCED_FACE('',(#1271,#603),#5609,.F.);
#5920=ADVANCED_FACE('',(#1272),#464,.T.);
#5921=ADVANCED_FACE('',(#1273,#604),#5610,.F.);
#5922=ADVANCED_FACE('',(#1274),#465,.T.);
#5923=ADVANCED_FACE('',(#1275,#605),#5611,.T.);
#6024=CLOSED_SHELL('',(#5890,#5891,#5892,#5893,#5894,#5895,#5896,#5897,
#5898,#5899,#5900,#5901,#5902,#5903,#5904,#5905,#5906,#5907,#5908,#5909,
#5910,#5911,#5912,#5913));
#6703=AXIS2_PLACEMENT_3D('',#11193,#8213,#8214);
#6704=AXIS2_PLACEMENT_3D('',#11194,#8215,#8216);
#6705=AXIS2_PLACEMENT_3D('',#11202,#8220,#8221);
#6706=AXIS2_PLACEMENT_3D('',#11203,#8222,#8223);
#6707=AXIS2_PLACEMENT_3D('',#11205,#8224,#8225);
#6708=AXIS2_PLACEMENT_3D('',#11207,#8226,#8227);
#6709=AXIS2_PLACEMENT_3D('',#11209,#8229,#8230);
#6710=AXIS2_PLACEMENT_3D('',#11216,#8234,#8235);
#6711=AXIS2_PLACEMENT_3D('',#11218,#8236,#8237);
#6712=AXIS2_PLACEMENT_3D('',#11220,#8238,#8239);
#6713=AXIS2_PLACEMENT_3D('',#11221,#8240,#8241);
#6714=AXIS2_PLACEMENT_3D('',#11261,#8243,#8244);
#6715=AXIS2_PLACEMENT_3D('',#11263,#8245,#8246);
#6716=AXIS2_PLACEMENT_3D('',#11266,#8248,#8249);
#6717=AXIS2_PLACEMENT_3D('',#11305,#8250,#8251);
#6718=AXIS2_PLACEMENT_3D('',#11307,#8252,#8253);
#6719=AXIS2_PLACEMENT_3D('',#11309,#8254,#8255);
#6720=AXIS2_PLACEMENT_3D('',#11311,#8256,#8257);
#6721=AXIS2_PLACEMENT_3D('',#11313,#8258,#8259);
#6722=AXIS2_PLACEMENT_3D('',#11314,#8260,#8261);
#6723=AXIS2_PLACEMENT_3D('',#11318,#8263,#8264);
#6724=AXIS2_PLACEMENT_3D('',#11319,#8265,#8266);
#6725=AXIS2_PLACEMENT_3D('',#11320,#8267,#8268);
#6726=AXIS2_PLACEMENT_3D('',#11322,#8269,#8270);
#6727=AXIS2_PLACEMENT_3D('',#11323,#8271,#8272);
#6728=AXIS2_PLACEMENT_3D('',#11324,#8273,#8274);
#6729=AXIS2_PLACEMENT_3D('',#11326,#8275,#8276);
#6730=AXIS2_PLACEMENT_3D('',#11328,#8277,#8278);
#6731=AXIS2_PLACEMENT_3D('',#11330,#8279,#8280);
#6732=AXIS2_PLACEMENT_3D('',#11332,#8281,#8282);
#6733=AXIS2_PLACEMENT_3D('',#11333,#8283,#8284);
#6734=AXIS2_PLACEMENT_3D('',#11335,#8286,#8287);
#6735=AXIS2_PLACEMENT_3D('',#11337,#8289,#8290);
#6736=AXIS2_PLACEMENT_3D('',#11339,#8292,#8293);
#6737=AXIS2_PLACEMENT_3D('',#11341,#8294,#8295);
#6738=AXIS2_PLACEMENT_3D('',#11343,#8296,#8297);
#6739=AXIS2_PLACEMENT_3D('',#11344,#8298,#8299);
#6740=AXIS2_PLACEMENT_3D('',#11345,#8300,#8301);
#6741=AXIS2_PLACEMENT_3D('',#11349,#8303,#8304);
#6742=AXIS2_PLACEMENT_3D('',#11352,#8306,#8307);
#6743=AXIS2_PLACEMENT_3D('',#11389,#8309,#8310);
#6744=AXIS2_PLACEMENT_3D('',#11391,#8312,#8313);
#6745=AXIS2_PLACEMENT_3D('',#11394,#8314,#8315);
#6746=AXIS2_PLACEMENT_3D('',#11403,#8316,#8317);
#6747=AXIS2_PLACEMENT_3D('',#11406,#8320,#8321);
#6748=AXIS2_PLACEMENT_3D('',#11407,#8322,#8323);
#6749=AXIS2_PLACEMENT_3D('',#11408,#8324,#8325);
#6750=AXIS2_PLACEMENT_3D('',#11409,#8326,#8327);
#6751=AXIS2_PLACEMENT_3D('',#11411,#8329,#8330);
#6752=AXIS2_PLACEMENT_3D('',#11412,#8331,#8332);
#6753=AXIS2_PLACEMENT_3D('',#11413,#8333,#8334);
#6754=AXIS2_PLACEMENT_3D('',#11415,#8335,#8336);
#6755=AXIS2_PLACEMENT_3D('',#11417,#8338,#8339);
#6756=AXIS2_PLACEMENT_3D('',#11418,#8340,#8341);
#6757=AXIS2_PLACEMENT_3D('',#11420,#8342,#8343);
#6758=AXIS2_PLACEMENT_3D('',#11423,#8345,#8346);
#6759=AXIS2_PLACEMENT_3D('',#11424,#8347,#8348);
#6760=AXIS2_PLACEMENT_3D('',#11426,#8349,#8350);
#6761=AXIS2_PLACEMENT_3D('',#11427,#8351,#8352);
#6762=AXIS2_PLACEMENT_3D('',#11429,#8353,#8354);
#6763=AXIS2_PLACEMENT_3D('',#11432,#8356,#8357);
#6764=AXIS2_PLACEMENT_3D('',#11433,#8358,#8359);
#6765=AXIS2_PLACEMENT_3D('',#11435,#8360,#8361);
#6766=AXIS2_PLACEMENT_3D('',#11436,#8362,#8363);
#6767=AXIS2_PLACEMENT_3D('',#11438,#8364,#8365);
#6768=AXIS2_PLACEMENT_3D('',#11441,#8367,#8368);
#6769=AXIS2_PLACEMENT_3D('',#11442,#8369,#8370);
#6770=AXIS2_PLACEMENT_3D('',#11444,#8371,#8372);
#6771=AXIS2_PLACEMENT_3D('',#11445,#8373,#8374);
#6772=AXIS2_PLACEMENT_3D('',#11447,#8375,#8376);
#6773=AXIS2_PLACEMENT_3D('',#11450,#8378,#8379);
#6774=AXIS2_PLACEMENT_3D('',#11451,#8380,#8381);
#6775=AXIS2_PLACEMENT_3D('',#11453,#8382,#8383);
#6776=AXIS2_PLACEMENT_3D('',#11454,#8384,#8385);
#6777=AXIS2_PLACEMENT_3D('',#11456,#8386,#8387);
#6778=AXIS2_PLACEMENT_3D('',#11459,#8389,#8390);
#6779=AXIS2_PLACEMENT_3D('',#11460,#8391,#8392);
#6780=AXIS2_PLACEMENT_3D('',#11462,#8393,#8394);
#8213=DIRECTION('axis',(0.,0.,1.));
#8214=DIRECTION('refdir',(1.,0.,0.));
#8215=DIRECTION('center_axis',(0.,0.,-1.));
#8216=DIRECTION('ref_axis',(0.,-1.,0.));
#8217=DIRECTION('',(1.,0.,0.));
#8218=DIRECTION('',(0.,-1.,0.));
#8219=DIRECTION('',(-1.,0.,0.));
#8220=DIRECTION('center_axis',(0.,0.,1.));
#8221=DIRECTION('ref_axis',(0.,1.,0.));
#8222=DIRECTION('center_axis',(1.,0.,0.));
#8223=DIRECTION('ref_axis',(0.,0.,1.));
#8224=DIRECTION('center_axis',(1.,0.,0.));
#8225=DIRECTION('ref_axis',(0.,0.,1.));
#8226=DIRECTION('center_axis',(1.,0.,0.));
#8227=DIRECTION('ref_axis',(0.,0.,1.));
#8228=DIRECTION('',(1.,0.,0.));
#8229=DIRECTION('center_axis',(1.,0.,0.));
#8230=DIRECTION('ref_axis',(0.,-1.,0.));
#8231=DIRECTION('',(0.,0.,-1.));
#8232=DIRECTION('',(0.,1.,0.));
#8233=DIRECTION('',(0.,0.,1.));
#8234=DIRECTION('center_axis',(1.,0.,0.));
#8235=DIRECTION('ref_axis',(0.,1.,0.));
#8236=DIRECTION('center_axis',(1.,0.,0.));
#8237=DIRECTION('ref_axis',(0.,0.,-1.));
#8238=DIRECTION('center_axis',(1.,0.,0.));
#8239=DIRECTION('ref_axis',(0.,-1.,0.));
#8240=DIRECTION('center_axis',(1.,0.,0.));
#8241=DIRECTION('ref_axis',(0.,-1.,0.));
#8242=DIRECTION('',(1.,0.,0.));
#8243=DIRECTION('center_axis',(0.,0.,-1.));
#8244=DIRECTION('ref_axis',(0.,-1.,0.));
#8245=DIRECTION('center_axis',(0.,0.,-1.));
#8246=DIRECTION('ref_axis',(0.,1.,0.));
#8247=DIRECTION('',(0.,0.,-1.));
#8248=DIRECTION('center_axis',(0.,0.,-1.));
#8249=DIRECTION('ref_axis',(0.,1.,0.));
#8250=DIRECTION('center_axis',(0.,0.,-1.));
#8251=DIRECTION('ref_axis',(0.,-1.,0.));
#8252=DIRECTION('center_axis',(0.,0.,1.));
#8253=DIRECTION('ref_axis',(0.,-1.,0.));
#8254=DIRECTION('center_axis',(0.,0.,-1.));
#8255=DIRECTION('ref_axis',(1.,0.,0.));
#8256=DIRECTION('center_axis',(0.,0.,-1.));
#8257=DIRECTION('ref_axis',(1.,0.,0.));
#8258=DIRECTION('center_axis',(0.,0.,-1.));
#8259=DIRECTION('ref_axis',(1.,0.,0.));
#8260=DIRECTION('center_axis',(0.,0.,-1.));
#8261=DIRECTION('ref_axis',(0.,-1.,0.));
#8262=DIRECTION('',(0.,0.,1.));
#8263=DIRECTION('center_axis',(0.,0.,-1.));
#8264=DIRECTION('ref_axis',(0.,1.,0.));
#8265=DIRECTION('center_axis',(0.,0.,-1.));
#8266=DIRECTION('ref_axis',(0.,1.,0.));
#8267=DIRECTION('center_axis',(0.,0.,-1.));
#8268=DIRECTION('ref_axis',(-0.0100738296067504,0.999949257691136,0.));
#8269=DIRECTION('center_axis',(-0.999949257691136,-0.0100738296067502,0.));
#8270=DIRECTION('ref_axis',(0.0100738296067502,-0.999949257691136,0.));
#8271=DIRECTION('center_axis',(0.,0.,-1.));
#8272=DIRECTION('ref_axis',(0.,1.,0.));
#8273=DIRECTION('center_axis',(0.,0.,-1.));
#8274=DIRECTION('ref_axis',(0.,-1.,0.));
#8275=DIRECTION('center_axis',(0.,0.,-1.));
#8276=DIRECTION('ref_axis',(1.,0.,0.));
#8277=DIRECTION('center_axis',(0.,0.,-1.));
#8278=DIRECTION('ref_axis',(1.,0.,0.));
#8279=DIRECTION('center_axis',(0.,0.,1.));
#8280=DIRECTION('ref_axis',(0.,1.,0.));
#8281=DIRECTION('center_axis',(0.,0.,-1.));
#8282=DIRECTION('ref_axis',(1.,0.,0.));
#8283=DIRECTION('center_axis',(0.,0.,-1.));
#8284=DIRECTION('ref_axis',(1.,0.,0.));
#8285=DIRECTION('',(0.,0.,-1.));
#8286=DIRECTION('center_axis',(0.,0.,-1.));
#8287=DIRECTION('ref_axis',(1.,0.,0.));
#8288=DIRECTION('',(0.,0.,-1.));
#8289=DIRECTION('center_axis',(0.,0.,-1.));
#8290=DIRECTION('ref_axis',(1.,0.,0.));
#8291=DIRECTION('',(0.,0.,-1.));
#8292=DIRECTION('center_axis',(0.,0.,-1.));
#8293=DIRECTION('ref_axis',(0.0208019280434405,0.999783616483925,0.));
#8294=DIRECTION('center_axis',(0.999783616483925,-0.0208019280434406,0.));
#8295=DIRECTION('ref_axis',(-0.0208019280434406,-0.999783616483925,0.));
#8296=DIRECTION('center_axis',(0.,0.,1.));
#8297=DIRECTION('ref_axis',(0.,1.,0.));
#8298=DIRECTION('center_axis',(0.,0.,1.));
#8299=DIRECTION('ref_axis',(0.,1.,0.));
#8300=DIRECTION('center_axis',(0.,0.,-1.));
#8301=DIRECTION('ref_axis',(0.,-1.,0.));
#8302=DIRECTION('',(0.,0.,1.));
#8303=DIRECTION('center_axis',(0.,0.,-1.));
#8304=DIRECTION('ref_axis',(0.,1.,0.));
#8305=DIRECTION('',(7.876565977693E-12,-1.341720385588E-11,1.));
#8306=DIRECTION('center_axis',(0.,0.,1.));
#8307=DIRECTION('ref_axis',(0.,1.,0.));
#8308=DIRECTION('',(-2.869570000055E-11,-1.341720385588E-11,-1.));
#8309=DIRECTION('center_axis',(1.,0.,0.));
#8310=DIRECTION('ref_axis',(0.,-1.,0.));
#8311=DIRECTION('',(1.,0.,0.));
#8312=DIRECTION('center_axis',(0.,0.,-1.));
#8313=DIRECTION('ref_axis',(0.999999999999998,-7.01586580949265E-8,0.));
#8314=DIRECTION('center_axis',(0.,0.,1.));
#8315=DIRECTION('ref_axis',(0.298065387468285,-0.954545454545451,0.));
#8316=DIRECTION('center_axis',(0.,0.,-1.));
#8317=DIRECTION('ref_axis',(0.,1.,0.));
#8318=DIRECTION('',(-1.,-3.471931990194E-12,0.));
#8319=DIRECTION('',(-1.,0.,0.));
#8320=DIRECTION('center_axis',(0.,-1.,0.));
#8321=DIRECTION('ref_axis',(0.,0.,-1.));
#8322=DIRECTION('center_axis',(0.,0.,-1.));
#8323=DIRECTION('ref_axis',(-1.,-1.05025155239247E-11,0.));
#8324=DIRECTION('center_axis',(-1.,0.,0.));
#8325=DIRECTION('ref_axis',(0.,0.,1.));
#8326=DIRECTION('center_axis',(-1.,0.,0.));
#8327=DIRECTION('ref_axis',(0.,0.,1.));
#8328=DIRECTION('',(-1.,0.,0.));
#8329=DIRECTION('center_axis',(0.,1.,0.));
#8330=DIRECTION('ref_axis',(0.,0.,1.));
#8331=DIRECTION('center_axis',(0.,0.,-1.));
#8332=DIRECTION('ref_axis',(0.,-1.,0.));
#8333=DIRECTION('center_axis',(1.,0.,0.));
#8334=DIRECTION('ref_axis',(0.,0.,1.));
#8335=DIRECTION('center_axis',(1.,0.,0.));
#8336=DIRECTION('ref_axis',(0.,0.,-1.));
#8337=DIRECTION('',(-1.,0.,0.));
#8338=DIRECTION('center_axis',(1.,0.,0.));
#8339=DIRECTION('ref_axis',(0.,0.,1.));
#8340=DIRECTION('center_axis',(0.,0.,-1.));
#8341=DIRECTION('ref_axis',(-1.,0.,0.));
#8342=DIRECTION('center_axis',(0.,0.,-1.));
#8343=DIRECTION('ref_axis',(1.,0.,0.));
#8344=DIRECTION('',(0.,0.,1.));
#8345=DIRECTION('center_axis',(0.,0.,-1.));
#8346=DIRECTION('ref_axis',(1.,0.,0.));
#8347=DIRECTION('center_axis',(0.,0.,-1.));
#8348=DIRECTION('ref_axis',(-1.,0.,0.));
#8349=DIRECTION('center_axis',(0.,0.,1.));
#8350=DIRECTION('ref_axis',(1.,0.,0.));
#8351=DIRECTION('center_axis',(0.,0.,-1.));
#8352=DIRECTION('ref_axis',(-1.,0.,0.));
#8353=DIRECTION('center_axis',(0.,0.,-1.));
#8354=DIRECTION('ref_axis',(1.,0.,0.));
#8355=DIRECTION('',(0.,0.,1.));
#8356=DIRECTION('center_axis',(0.,0.,-1.));
#8357=DIRECTION('ref_axis',(1.,0.,0.));
#8358=DIRECTION('center_axis',(0.,0.,-1.));
#8359=DIRECTION('ref_axis',(-1.,0.,0.));
#8360=DIRECTION('center_axis',(0.,0.,1.));
#8361=DIRECTION('ref_axis',(1.,0.,0.));
#8362=DIRECTION('center_axis',(0.,0.,-1.));
#8363=DIRECTION('ref_axis',(-1.,0.,0.));
#8364=DIRECTION('center_axis',(0.,0.,-1.));
#8365=DIRECTION('ref_axis',(1.,0.,0.));
#8366=DIRECTION('',(0.,0.,1.));
#8367=DIRECTION('center_axis',(0.,0.,-1.));
#8368=DIRECTION('ref_axis',(1.,0.,0.));
#8369=DIRECTION('center_axis',(0.,0.,-1.));
#8370=DIRECTION('ref_axis',(-1.,0.,0.));
#8371=DIRECTION('center_axis',(0.,0.,1.));
#8372=DIRECTION('ref_axis',(1.,0.,0.));
#8373=DIRECTION('center_axis',(1.,0.,0.));
#8374=DIRECTION('ref_axis',(0.,1.,0.));
#8375=DIRECTION('center_axis',(1.,0.,0.));
#8376=DIRECTION('ref_axis',(0.,-1.,0.));
#8377=DIRECTION('',(-1.,0.,0.));
#8378=DIRECTION('center_axis',(1.,0.,0.));
#8379=DIRECTION('ref_axis',(0.,-1.,0.));
#8380=DIRECTION('center_axis',(1.,0.,0.));
#8381=DIRECTION('ref_axis',(0.,1.,0.));
#8382=DIRECTION('center_axis',(-1.,0.,0.));
#8383=DIRECTION('ref_axis',(0.,-1.,0.));
#8384=DIRECTION('center_axis',(1.,0.,0.));
#8385=DIRECTION('ref_axis',(0.,1.,0.));
#8386=DIRECTION('center_axis',(1.,0.,0.));
#8387=DIRECTION('ref_axis',(0.,-1.,0.));
#8388=DIRECTION('',(-1.,0.,0.));
#8389=DIRECTION('center_axis',(1.,0.,0.));
#8390=DIRECTION('ref_axis',(0.,-1.,0.));
#8391=DIRECTION('center_axis',(1.,0.,0.));
#8392=DIRECTION('ref_axis',(0.,1.,0.));
#8393=DIRECTION('center_axis',(-1.,0.,0.));
#8394=DIRECTION('ref_axis',(0.,-1.,0.));
#11193=CARTESIAN_POINT('',(0.,0.,0.));
#11194=CARTESIAN_POINT('Origin',(0.,0.,0.));
#11195=CARTESIAN_POINT('',(0.,-10.,0.));
#11196=CARTESIAN_POINT('',(14.,-10.,0.));
#11197=CARTESIAN_POINT('',(0.,-10.,0.));
#11198=CARTESIAN_POINT('',(14.,10.,0.));
#11199=CARTESIAN_POINT('',(14.,10.,0.));
#11200=CARTESIAN_POINT('',(0.,10.,0.));
#11201=CARTESIAN_POINT('',(14.,10.,0.));
#11202=CARTESIAN_POINT('Origin',(0.,0.,0.));
#11203=CARTESIAN_POINT('Origin',(-0.133704,-10.,-0.5));
#11204=CARTESIAN_POINT('',(14.,-10.5,-0.5));
#11205=CARTESIAN_POINT('Origin',(14.,-10.,-0.5));
#11206=CARTESIAN_POINT('',(2.205697222091E-10,-10.5,-0.5));
#11207=CARTESIAN_POINT('Origin',(0.,-10.,-0.5));
#11208=CARTESIAN_POINT('',(2.205697222091E-10,-10.5,-0.5));
#11209=CARTESIAN_POINT('Origin',(14.,0.,0.));
#11210=CARTESIAN_POINT('',(14.,-10.5,-28.));
#11211=CARTESIAN_POINT('',(14.,-10.5,-0.5));
#11212=CARTESIAN_POINT('',(14.,10.5,-28.));
#11213=CARTESIAN_POINT('',(14.,-10.5,-28.));
#11214=CARTESIAN_POINT('',(14.,10.5,-0.5));
#11215=CARTESIAN_POINT('',(14.,10.5,-28.));
#11216=CARTESIAN_POINT('Origin',(14.,10.,-0.5));
#11217=CARTESIAN_POINT('',(14.,0.,-24.));
#11218=CARTESIAN_POINT('Origin',(14.,0.,-22.));
#11219=CARTESIAN_POINT('',(14.,1.75,-7.));
#11220=CARTESIAN_POINT('Origin',(14.,0.,-7.));
#11221=CARTESIAN_POINT('Origin',(0.,0.,-7.));
#11222=CARTESIAN_POINT('',(7.806247497998,-1.75,-7.));
#11223=CARTESIAN_POINT('',(7.806247497998,1.75,-7.));
#11224=CARTESIAN_POINT('Ctrl Pts',(7.806247497998,-1.75,-7.));
#11225=CARTESIAN_POINT('Ctrl Pts',(7.806247497998,-1.75,-7.22051202732056));
#11226=CARTESIAN_POINT('Ctrl Pts',(7.81656151369615,-1.70578419252538,-7.45521537354111));
#11227=CARTESIAN_POINT('Ctrl Pts',(7.85345055027074,-1.52697344069322,-7.8861563440924));
#11228=CARTESIAN_POINT('Ctrl Pts',(7.8794534058773,-1.3924155896664,-8.08245814448651));
#11229=CARTESIAN_POINT('Ctrl Pts',(7.9279795931108,-1.08247066684372,-8.39240306730919));
#11230=CARTESIAN_POINT('Ctrl Pts',(7.95370820844925,-0.886163584469686,
-8.52697071250845));
#11231=CARTESIAN_POINT('Ctrl Pts',(7.98996554209154,-0.455204126605999,
-8.7057885831527));
#11232=CARTESIAN_POINT('Ctrl Pts',(8.,-0.220494209840019,-8.75));
#11233=CARTESIAN_POINT('Ctrl Pts',(8.,0.220494209840019,-8.75));
#11234=CARTESIAN_POINT('Ctrl Pts',(7.98996554209154,0.455204126605999,-8.7057885831527));
#11235=CARTESIAN_POINT('Ctrl Pts',(7.95370820844925,0.886163584469686,-8.52697071250845));
#11236=CARTESIAN_POINT('Ctrl Pts',(7.9279795931108,1.08247066684372,-8.39240306730919));
#11237=CARTESIAN_POINT('Ctrl Pts',(7.8794534058773,1.3924155896664,-8.08245814448651));
#11238=CARTESIAN_POINT('Ctrl Pts',(7.85345055027074,1.52697344069322,-7.8861563440924));
#11239=CARTESIAN_POINT('Ctrl Pts',(7.81656151369615,1.70578419252538,-7.45521537354111));
#11240=CARTESIAN_POINT('Ctrl Pts',(7.806247497998,1.75,-7.22051202732056));
#11241=CARTESIAN_POINT('Ctrl Pts',(7.806247497998,1.75,-7.));
#11242=CARTESIAN_POINT('Ctrl Pts',(7.806247497998,1.75,-7.));
#11243=CARTESIAN_POINT('Ctrl Pts',(7.806247497998,1.75,-6.77948797267944));
#11244=CARTESIAN_POINT('Ctrl Pts',(7.81656151369615,1.70578419252538,-6.5447846264589));
#11245=CARTESIAN_POINT('Ctrl Pts',(7.85345055027074,1.52697344069322,-6.1138436559076));
#11246=CARTESIAN_POINT('Ctrl Pts',(7.8794534058773,1.3924155896664,-5.91754185551349));
#11247=CARTESIAN_POINT('Ctrl Pts',(7.9279795931108,1.08247066684372,-5.60759693269081));
#11248=CARTESIAN_POINT('Ctrl Pts',(7.95370820844925,0.886163584469687,-5.47302928749155));
#11249=CARTESIAN_POINT('Ctrl Pts',(7.98996554209154,0.455204126606001,-5.2942114168473));
#11250=CARTESIAN_POINT('Ctrl Pts',(8.,0.220494209840019,-5.25));
#11251=CARTESIAN_POINT('Ctrl Pts',(8.,-0.220494209840019,-5.25));
#11252=CARTESIAN_POINT('Ctrl Pts',(7.98996554209154,-0.455204126606001,
-5.2942114168473));
#11253=CARTESIAN_POINT('Ctrl Pts',(7.95370820844925,-0.886163584469688,
-5.47302928749155));
#11254=CARTESIAN_POINT('Ctrl Pts',(7.9279795931108,-1.08247066684372,-5.60759693269081));
#11255=CARTESIAN_POINT('Ctrl Pts',(7.8794534058773,-1.3924155896664,-5.91754185551349));
#11256=CARTESIAN_POINT('Ctrl Pts',(7.85345055027074,-1.52697344069322,-6.1138436559076));
#11257=CARTESIAN_POINT('Ctrl Pts',(7.81656151369615,-1.70578419252538,-6.5447846264589));
#11258=CARTESIAN_POINT('Ctrl Pts',(7.806247497998,-1.75,-6.77948797267944));
#11259=CARTESIAN_POINT('Ctrl Pts',(7.806247497998,-1.75,-7.));
#11260=CARTESIAN_POINT('',(0.,1.75,-7.));
#11261=CARTESIAN_POINT('Origin',(0.,0.,-55.));
#11262=CARTESIAN_POINT('',(0.,8.,-3.));
#11263=CARTESIAN_POINT('Origin',(0.,0.,-3.));
#11264=CARTESIAN_POINT('',(0.,8.,-55.));
#11265=CARTESIAN_POINT('',(9.79717439317883E-16,8.,-55.));
#11266=CARTESIAN_POINT('Origin',(0.,0.,-55.));
#11267=CARTESIAN_POINT('',(7.745966692415,-2.,-48.));
#11268=CARTESIAN_POINT('',(7.74596669241483,2.,-48.));
#11269=CARTESIAN_POINT('Ctrl Pts',(7.74596669241483,-2.,-48.));
#11270=CARTESIAN_POINT('Ctrl Pts',(7.74596669241483,-2.,-48.2522988213568));
#11271=CARTESIAN_POINT('Ctrl Pts',(7.75957726931369,-1.94935810817991,-48.520643416021));
#11272=CARTESIAN_POINT('Ctrl Pts',(7.8080895555786,-1.74492797023227,-49.0130613700609));
#11273=CARTESIAN_POINT('Ctrl Pts',(7.84222121032682,-1.59119421565163,-49.2372329090946));
#11274=CARTESIAN_POINT('Ctrl Pts',(7.90579009335489,-1.23725765414306,-49.5911694706031));
#11275=CARTESIAN_POINT('Ctrl Pts',(7.93945007560674,-1.01307580920409,-49.7449225186146));
#11276=CARTESIAN_POINT('Ctrl Pts',(7.98687320195912,-0.52062131163299,-49.9493667420601));
#11277=CARTESIAN_POINT('Ctrl Pts',(8.,-0.252263545486473,-50.));
#11278=CARTESIAN_POINT('Ctrl Pts',(8.,0.252263545486474,-50.));
#11279=CARTESIAN_POINT('Ctrl Pts',(7.98687320195912,0.520621311632991,-49.9493667420601));
#11280=CARTESIAN_POINT('Ctrl Pts',(7.93945007560674,1.01307580920409,-49.7449225186146));
#11281=CARTESIAN_POINT('Ctrl Pts',(7.90579009335489,1.23725765414306,-49.5911694706031));
#11282=CARTESIAN_POINT('Ctrl Pts',(7.84222121032682,1.59119421565164,-49.2372329090946));
#11283=CARTESIAN_POINT('Ctrl Pts',(7.8080895555786,1.74492797023227,-49.0130613700609));
#11284=CARTESIAN_POINT('Ctrl Pts',(7.75957726931369,1.94935810817991,-48.520643416021));
#11285=CARTESIAN_POINT('Ctrl Pts',(7.74596669241483,2.,-48.2522988213568));
#11286=CARTESIAN_POINT('Ctrl Pts',(7.74596669241483,2.,-48.));
#11287=CARTESIAN_POINT('Ctrl Pts',(7.74596669241483,2.,-48.));
#11288=CARTESIAN_POINT('Ctrl Pts',(7.74596669241483,2.,-47.7477011786432));
#11289=CARTESIAN_POINT('Ctrl Pts',(7.75957726931369,1.94935810817991,-47.479356583979));
#11290=CARTESIAN_POINT('Ctrl Pts',(7.8080895555786,1.74492797023228,-46.9869386299392));
#11291=CARTESIAN_POINT('Ctrl Pts',(7.84222121032682,1.59119421565164,-46.7627670909054));
#11292=CARTESIAN_POINT('Ctrl Pts',(7.90579009335489,1.23725765414306,-46.4088305293969));
#11293=CARTESIAN_POINT('Ctrl Pts',(7.93945007560674,1.01307580920409,-46.2550774813855));
#11294=CARTESIAN_POINT('Ctrl Pts',(7.98687320195912,0.520621311632997,-46.0506332579399));
#11295=CARTESIAN_POINT('Ctrl Pts',(8.,0.252263545486474,-46.));
#11296=CARTESIAN_POINT('Ctrl Pts',(8.,-0.252263545486474,-46.));
#11297=CARTESIAN_POINT('Ctrl Pts',(7.98687320195912,-0.520621311632997,
-46.0506332579399));
#11298=CARTESIAN_POINT('Ctrl Pts',(7.93945007560674,-1.01307580920409,-46.2550774813855));
#11299=CARTESIAN_POINT('Ctrl Pts',(7.90579009335489,-1.23725765414306,-46.4088305293969));
#11300=CARTESIAN_POINT('Ctrl Pts',(7.84222121032682,-1.59119421565164,-46.7627670909054));
#11301=CARTESIAN_POINT('Ctrl Pts',(7.8080895555786,-1.74492797023227,-46.9869386299391));
#11302=CARTESIAN_POINT('Ctrl Pts',(7.75957726931369,-1.94935810817991,-47.479356583979));
#11303=CARTESIAN_POINT('Ctrl Pts',(7.74596669241483,-2.,-47.7477011786432));
#11304=CARTESIAN_POINT('Ctrl Pts',(7.74596669241483,-2.,-48.));
#11305=CARTESIAN_POINT('Origin',(0.,0.,-55.));
#11306=CARTESIAN_POINT('',(0.,16.,-55.));
#11307=CARTESIAN_POINT('Origin',(0.,0.,-55.));
#11308=CARTESIAN_POINT('',(-14.25,0.,-55.));
#11309=CARTESIAN_POINT('Origin',(-13.,0.,-55.));
#11310=CARTESIAN_POINT('',(5.678203230276,-11.,-55.));
#11311=CARTESIAN_POINT('Origin',(6.928203230276,-11.,-55.));
#11312=CARTESIAN_POINT('',(5.678203230276,11.,-55.));
#11313=CARTESIAN_POINT('Origin',(6.928203230276,11.,-55.));
#11314=CARTESIAN_POINT('Origin',(0.,0.,2.75));
#11315=CARTESIAN_POINT('',(0.,16.,-51.5));
#11316=CARTESIAN_POINT('',(1.95943487863577E-15,16.,2.75));
#11317=CARTESIAN_POINT('',(0.161181273708004,-15.9991881230582,-51.5));
#11318=CARTESIAN_POINT('Origin',(0.,0.,-51.5));
#11319=CARTESIAN_POINT('Origin',(0.,0.,-51.5));
#11320=CARTESIAN_POINT('Origin',(0.,0.,-51.5));
#11321=CARTESIAN_POINT('',(0.156144358904629,-15.4992134942126,-51.));
#11322=CARTESIAN_POINT('Origin',(0.156144358904629,-15.4992134942126,-51.5));
#11323=CARTESIAN_POINT('Origin',(0.,0.,-51.));
#11324=CARTESIAN_POINT('Origin',(0.,0.,-51.));
#11325=CARTESIAN_POINT('',(5.678203230276,-11.,-51.));
#11326=CARTESIAN_POINT('Origin',(6.928203230276,-11.,-51.));
#11327=CARTESIAN_POINT('',(5.678203230276,11.,-51.));
#11328=CARTESIAN_POINT('Origin',(6.928203230276,11.,-51.));
#11329=CARTESIAN_POINT('',(-0.228821208477847,-10.9976197813232,-51.));
#11330=CARTESIAN_POINT('Origin',(0.,0.,-51.));
#11331=CARTESIAN_POINT('',(-14.25,0.,-51.));
#11332=CARTESIAN_POINT('Origin',(-13.,0.,-51.));
#11333=CARTESIAN_POINT('Origin',(-13.,0.,-55.));
#11334=CARTESIAN_POINT('',(-14.25,1.53080849893419E-16,-55.));
#11335=CARTESIAN_POINT('Origin',(6.928203230276,-11.,-55.));
#11336=CARTESIAN_POINT('',(5.678203230276,-11.,-55.));
#11337=CARTESIAN_POINT('Origin',(6.928203230276,11.,-55.));
#11338=CARTESIAN_POINT('',(5.678203230276,11.,-55.));
#11339=CARTESIAN_POINT('Origin',(0.,0.,-50.5));
#11340=CARTESIAN_POINT('',(-0.218420244456127,-10.4977279730812,-50.5));
#11341=CARTESIAN_POINT('Origin',(-0.228821208477847,-10.9976197813232,-50.5));
#11342=CARTESIAN_POINT('',(0.,10.5,-50.5));
#11343=CARTESIAN_POINT('Origin',(0.,0.,-50.5));
#11344=CARTESIAN_POINT('Origin',(0.,0.,-50.5));
#11345=CARTESIAN_POINT('Origin',(0.,0.,2.75));
#11346=CARTESIAN_POINT('',(0.,10.4999999995,-28.5));
#11347=CARTESIAN_POINT('',(1.28587913910472E-15,10.5,2.75));
#11348=CARTESIAN_POINT('',(2.58748336760221E-14,-10.4999999995,-28.5));
#11349=CARTESIAN_POINT('Origin',(0.,0.,-28.5));
#11350=CARTESIAN_POINT('',(2.587483367663E-14,-10.49999999962,-28.5));
#11351=CARTESIAN_POINT('',(0.,10.5,-0.5));
#11352=CARTESIAN_POINT('Origin',(0.,0.,-0.5));
#11353=CARTESIAN_POINT('',(8.034813416777E-10,10.5,-0.5));
#11354=CARTESIAN_POINT('',(10.30776406404,2.,-48.));
#11355=CARTESIAN_POINT('Ctrl Pts',(10.3077640640442,-2.,-48.));
#11356=CARTESIAN_POINT('Ctrl Pts',(10.3077640640442,-2.,-47.7482070465008));
#11357=CARTESIAN_POINT('Ctrl Pts',(10.3179460772103,-1.94955285220986,-47.4800636214909));
#11358=CARTESIAN_POINT('Ctrl Pts',(10.3544601248255,-1.74525726713758,-46.9874944768476));
#11359=CARTESIAN_POINT('Ctrl Pts',(10.380236242486,-1.59144134502885,-46.7630142202827));
#11360=CARTESIAN_POINT('Ctrl Pts',(10.4284146976182,-1.2369939207975,-46.4085667960513));
#11361=CARTESIAN_POINT('Ctrl Pts',(10.4539852161582,-1.01251019566121,-46.2547444939347));
#11362=CARTESIAN_POINT('Ctrl Pts',(10.4900265771226,-0.519929037363746,
-46.050444279888));
#11363=CARTESIAN_POINT('Ctrl Pts',(10.5,-0.251781387216632,-46.));
#11364=CARTESIAN_POINT('Ctrl Pts',(10.5,0.251781387216631,-46.));
#11365=CARTESIAN_POINT('Ctrl Pts',(10.4900265771226,0.519929037363749,-46.050444279888));
#11366=CARTESIAN_POINT('Ctrl Pts',(10.4539852161582,1.01251019566121,-46.2547444939347));
#11367=CARTESIAN_POINT('Ctrl Pts',(10.4284146976182,1.2369939207975,-46.4085667960513));
#11368=CARTESIAN_POINT('Ctrl Pts',(10.380236242486,1.59144134502885,-46.7630142202827));
#11369=CARTESIAN_POINT('Ctrl Pts',(10.3544601248255,1.74525726713758,-46.9874944768476));
#11370=CARTESIAN_POINT('Ctrl Pts',(10.3179460772103,1.94955285220986,-47.4800636214909));
#11371=CARTESIAN_POINT('Ctrl Pts',(10.3077640640442,2.,-47.7482070465008));
#11372=CARTESIAN_POINT('Ctrl Pts',(10.3077640640442,2.,-48.2517929534992));
#11373=CARTESIAN_POINT('Ctrl Pts',(10.3179460772103,1.94955285220986,-48.5199363785091));
#11374=CARTESIAN_POINT('Ctrl Pts',(10.3544601248255,1.74525726713758,-49.0125055231524));
#11375=CARTESIAN_POINT('Ctrl Pts',(10.380236242486,1.59144134502885,-49.2369857797173));
#11376=CARTESIAN_POINT('Ctrl Pts',(10.4284146976182,1.2369939207975,-49.5914332039487));
#11377=CARTESIAN_POINT('Ctrl Pts',(10.4539852161582,1.01251019566121,-49.7452555060653));
#11378=CARTESIAN_POINT('Ctrl Pts',(10.4900265771226,0.519929037363747,-49.949555720112));
#11379=CARTESIAN_POINT('Ctrl Pts',(10.5,0.251781387216632,-50.));
#11380=CARTESIAN_POINT('Ctrl Pts',(10.5,-0.251781387216631,-50.));
#11381=CARTESIAN_POINT('Ctrl Pts',(10.4900265771226,-0.519929037363746,
-49.949555720112));
#11382=CARTESIAN_POINT('Ctrl Pts',(10.4539852161582,-1.01251019566121,-49.7452555060653));
#11383=CARTESIAN_POINT('Ctrl Pts',(10.4284146976182,-1.23699392079749,-49.5914332039487));
#11384=CARTESIAN_POINT('Ctrl Pts',(10.380236242486,-1.59144134502885,-49.2369857797173));
#11385=CARTESIAN_POINT('Ctrl Pts',(10.3544601248255,-1.74525726713758,-49.0125055231524));
#11386=CARTESIAN_POINT('Ctrl Pts',(10.3179460772103,-1.94955285220986,-48.5199363785091));
#11387=CARTESIAN_POINT('Ctrl Pts',(10.3077640640442,-2.,-48.2517929534992));
#11388=CARTESIAN_POINT('Ctrl Pts',(10.3077640640442,-2.,-48.));
#11389=CARTESIAN_POINT('Origin',(0.,0.,-48.));
#11390=CARTESIAN_POINT('',(0.,2.,-48.));
#11391=CARTESIAN_POINT('Origin',(0.,0.,-28.5));
#11392=CARTESIAN_POINT('',(3.27871926200197,-10.4999999995227,-28.));
#11393=CARTESIAN_POINT('',(3.27871926199412,10.4999999995103,-28.));
#11394=CARTESIAN_POINT('Origin',(0.,0.,-28.));
#11395=CARTESIAN_POINT('Ctrl Pts',(2.46987048725666E-14,-10.5,-28.5));
#11396=CARTESIAN_POINT('Ctrl Pts',(1.01790369883751,-10.5,-28.2778752023763));
#11397=CARTESIAN_POINT('Ctrl Pts',(2.23686160569662,-10.5,-28.));
#11398=CARTESIAN_POINT('Ctrl Pts',(3.27871925711855,-10.5,-28.));
#11399=CARTESIAN_POINT('Ctrl Pts',(3.27871925711855,10.5,-28.));
#11400=CARTESIAN_POINT('Ctrl Pts',(2.23686160569662,10.5,-27.9999999990974));
#11401=CARTESIAN_POINT('Ctrl Pts',(1.01790369883749,10.5,-28.2778752023763));
#11402=CARTESIAN_POINT('Ctrl Pts',(0.,10.5,-28.5));
#11403=CARTESIAN_POINT('Origin',(14.,-10.5,-28.));
#11404=CARTESIAN_POINT('',(14.,10.5,-28.));
#11405=CARTESIAN_POINT('',(14.,-10.5,-28.));
#11406=CARTESIAN_POINT('Origin',(14.,-10.5,0.));
#11407=CARTESIAN_POINT('Origin',(0.,0.,-0.5));
#11408=CARTESIAN_POINT('Origin',(0.,10.,-0.5));
#11409=CARTESIAN_POINT('Origin',(122.216,10.,-0.5));
#11410=CARTESIAN_POINT('',(14.,10.5,-0.5));
#11411=CARTESIAN_POINT('Origin',(14.,10.5,-28.));
#11412=CARTESIAN_POINT('Origin',(0.,0.,-3.));
#11413=CARTESIAN_POINT('Origin',(7.,0.,-22.));
#11414=CARTESIAN_POINT('',(49.,0.,-24.));
#11415=CARTESIAN_POINT('Origin',(49.,0.,-22.));
#11416=CARTESIAN_POINT('',(7.,2.44929359829471E-16,-24.));
#11417=CARTESIAN_POINT('Origin',(49.,0.,-22.));
#11418=CARTESIAN_POINT('Origin',(6.928203230276,-11.,-55.));
#11419=CARTESIAN_POINT('',(8.428203230276,-11.,-55.));
#11420=CARTESIAN_POINT('Origin',(6.928203230276,-11.,-55.));
#11421=CARTESIAN_POINT('',(8.428203230276,-11.,-51.));
#11422=CARTESIAN_POINT('',(8.428203230276,-11.,-55.));
#11423=CARTESIAN_POINT('Origin',(6.928203230276,-11.,-51.));
#11424=CARTESIAN_POINT('Origin',(6.928203230276,-11.,-51.));
#11425=CARTESIAN_POINT('',(5.678203230276,-11.,-51.));
#11426=CARTESIAN_POINT('Origin',(6.928203230276,-11.,-51.));
#11427=CARTESIAN_POINT('Origin',(-13.,0.,-55.));
#11428=CARTESIAN_POINT('',(-11.5,-1.83697019872103E-16,-55.));
#11429=CARTESIAN_POINT('Origin',(-13.,0.,-55.));
#11430=CARTESIAN_POINT('',(-11.5,-1.83697019872103E-16,-51.));
#11431=CARTESIAN_POINT('',(-11.5,-1.83697019872103E-16,-55.));
#11432=CARTESIAN_POINT('Origin',(-13.,0.,-51.));
#11433=CARTESIAN_POINT('Origin',(-13.,0.,-51.));
#11434=CARTESIAN_POINT('',(-14.25,0.,-51.));
#11435=CARTESIAN_POINT('Origin',(-13.,0.,-51.));
#11436=CARTESIAN_POINT('Origin',(6.928203230276,11.,-55.));
#11437=CARTESIAN_POINT('',(8.428203230276,11.,-55.));
#11438=CARTESIAN_POINT('Origin',(6.928203230276,11.,-55.));
#11439=CARTESIAN_POINT('',(8.428203230276,11.,-51.));
#11440=CARTESIAN_POINT('',(8.428203230276,11.,-55.));
#11441=CARTESIAN_POINT('Origin',(6.928203230276,11.,-51.));
#11442=CARTESIAN_POINT('Origin',(6.928203230276,11.,-51.));
#11443=CARTESIAN_POINT('',(5.678203230276,11.,-51.));
#11444=CARTESIAN_POINT('Origin',(6.928203230276,11.,-51.));
#11445=CARTESIAN_POINT('Origin',(14.,0.,-22.));
#11446=CARTESIAN_POINT('',(14.,-1.5,-22.));
#11447=CARTESIAN_POINT('Origin',(14.,0.,-22.));
#11448=CARTESIAN_POINT('',(9.,-1.5,-22.));
#11449=CARTESIAN_POINT('',(14.,-1.5,-22.));
#11450=CARTESIAN_POINT('Origin',(9.,0.,-22.));
#11451=CARTESIAN_POINT('Origin',(9.,0.,-22.));
#11452=CARTESIAN_POINT('',(9.,1.25,-22.));
#11453=CARTESIAN_POINT('Origin',(9.,0.,-22.));
#11454=CARTESIAN_POINT('Origin',(49.,0.,-22.));
#11455=CARTESIAN_POINT('',(49.,-1.75,-22.));
#11456=CARTESIAN_POINT('Origin',(49.,0.,-22.));
#11457=CARTESIAN_POINT('',(37.,-1.75,-22.));
#11458=CARTESIAN_POINT('',(49.,-1.75,-22.));
#11459=CARTESIAN_POINT('Origin',(37.,0.,-22.));
#11460=CARTESIAN_POINT('Origin',(37.,0.,-22.));
#11461=CARTESIAN_POINT('',(37.,2.,-22.));
#11462=CARTESIAN_POINT('Origin',(37.,0.,-22.));
#17081=UNCERTAINTY_MEASURE_WITH_UNIT(LENGTH_MEASURE(0.01),#17114,
'DISTANCE_ACCURACY_VALUE',
'Maximum model space distance between geometric entities at asserted c
onnectivities');
#17090=UNCERTAINTY_MEASURE_WITH_UNIT(LENGTH_MEASURE(0.01),#17114,
'DISTANCE_ACCURACY_VALUE',
'Maximum model space distance between geometric entities at asserted c
onnectivities');
#17104=(
GEOMETRIC_REPRESENTATION_CONTEXT(3)
GLOBAL_UNCERTAINTY_ASSIGNED_CONTEXT((#17081))
GLOBAL_UNIT_ASSIGNED_CONTEXT((#17114,#17116,#17117))
REPRESENTATION_CONTEXT('','3D')
);
#17113=(
GEOMETRIC_REPRESENTATION_CONTEXT(3)
GLOBAL_UNCERTAINTY_ASSIGNED_CONTEXT((#17090))
GLOBAL_UNIT_ASSIGNED_CONTEXT((#17114,#17116,#17117))
REPRESENTATION_CONTEXT('','3D')
);
#17114=(
LENGTH_UNIT()
NAMED_UNIT(*)
SI_UNIT(.MILLI.,.METRE.)
);
#17116=(
NAMED_UNIT(*)
PLANE_ANGLE_UNIT()
SI_UNIT($,.RADIAN.)
);
#17117=(
NAMED_UNIT(*)
SI_UNIT($,.STERADIAN.)
SOLID_ANGLE_UNIT()
);
#17131=SHAPE_DEFINITION_REPRESENTATION(#17162,#17197);
#17162=PRODUCT_DEFINITION_SHAPE('',$,#17220);
#17197=SHAPE_REPRESENTATION('',(#6703,#247,#248,#249,#250,#251),#17104);
#17206=PRODUCT_DEFINITION_CONTEXT('part definition',#17274,'design');
#17220=PRODUCT_DEFINITION('Cylinder','CYLINDER',#17242,#17206);
#17242=PRODUCT_DEFINITION_FORMATION('',$,#17289);
#17274=APPLICATION_CONTEXT(
'Core Data for Automotive Mechanical Design Process');
#17275=PRODUCT_CONTEXT('part definition',#17274,'mechanical');
#17289=PRODUCT('Cylinder','CYLINDER',$,(#17275));
#17298=PRESENTATION_STYLE_ASSIGNMENT((#17299));
#17299=SURFACE_STYLE_USAGE(.BOTH.,#17300);
#17300=SURFACE_SIDE_STYLE('',(#17301));
#17301=SURFACE_STYLE_FILL_AREA(#17302);
#17302=FILL_AREA_STYLE('Steel - Satin',(#17303));
#17303=FILL_AREA_STYLE_COLOUR('Steel - Satin',#17304);
#17304=COLOUR_RGB('Steel - Satin', 0.09019608, 0.27058824, 0.51372549);
ENDSEC;
END-ISO-10303-21;
